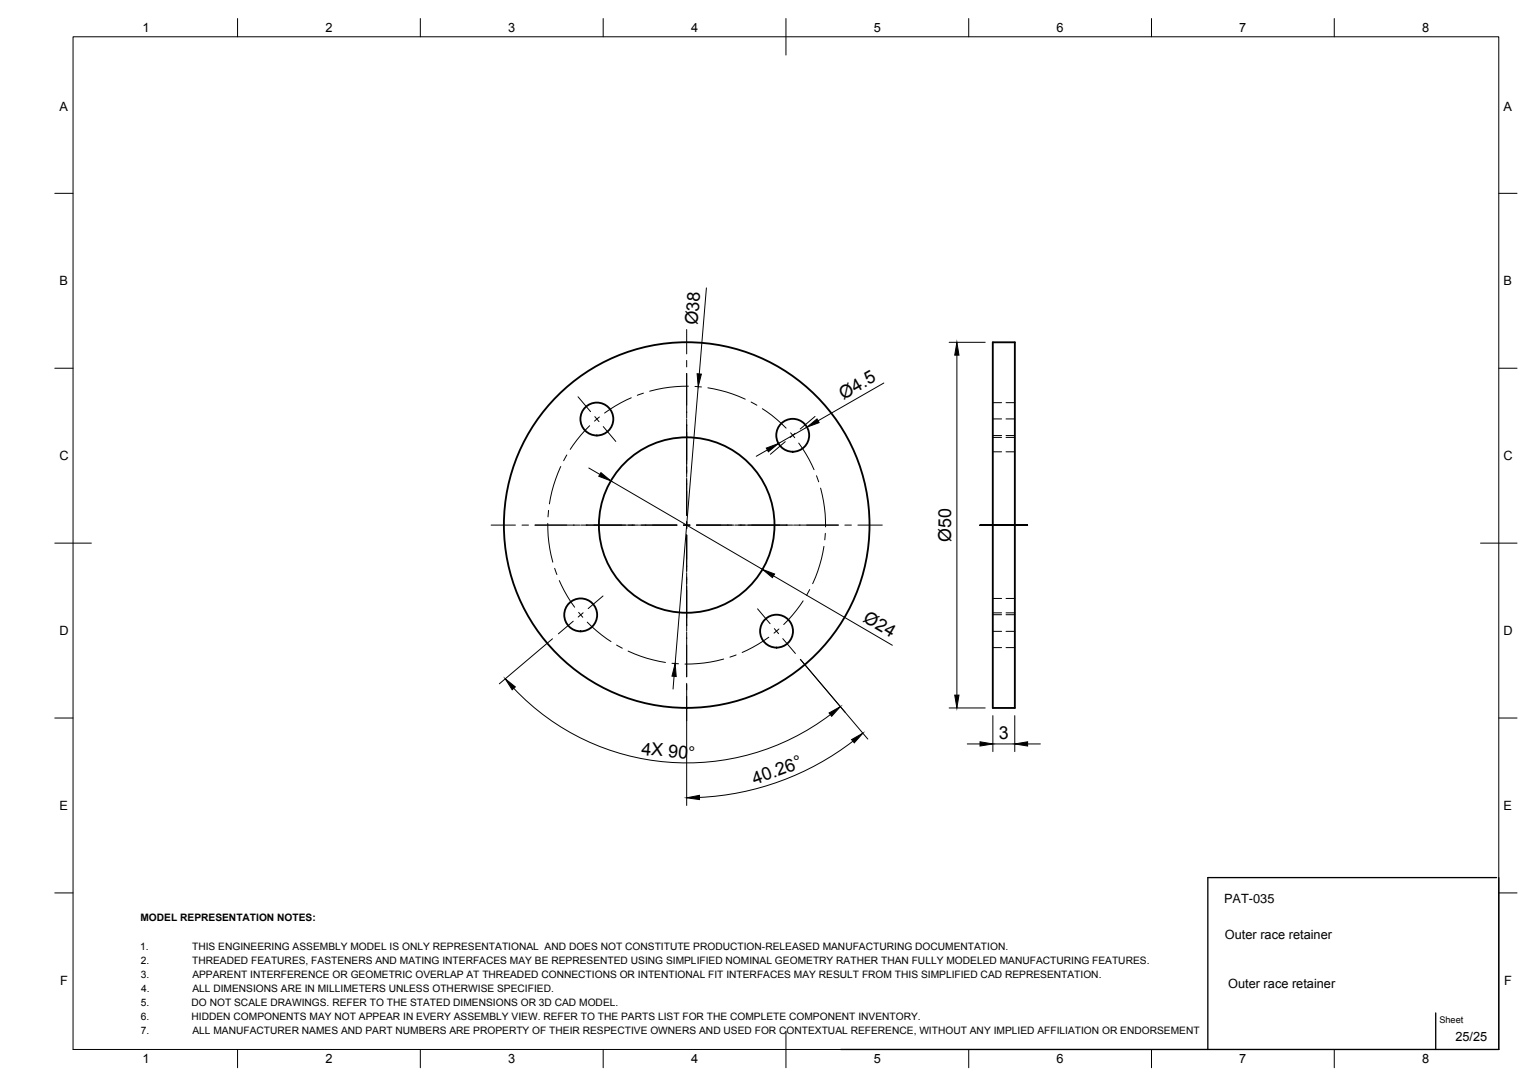
ISO-10303-21;
HEADER;
/* Generated by software containing ST-Developer
 * from STEP Tools, Inc. (www.steptools.com) 
 */

FILE_DESCRIPTION(
/* description */ ('Five-roller gravity conveyor'),
/* implementation_level */ '2;1');

FILE_NAME(
/* name */ 'Outer race retainer.step',
/* time_stamp */ '2026-10-29T15:36:43-07:00',
/* author */ (''),
/* organization */ (''),
/* preprocessor_version */ 'ST-DEVELOPER v20.2',
/* originating_system */ 'Autodesk Translation Framework v15.17.0.0',
/* authorisation */ '');

FILE_SCHEMA (('AUTOMOTIVE_DESIGN { 1 0 10303 214 3 1 1 }'));
ENDSEC;

DATA;
#10=MECHANICAL_DESIGN_GEOMETRIC_PRESENTATION_REPRESENTATION('',(#336),#7806);
#292=SHAPE_REPRESENTATION_RELATIONSHIP('SRR','None',#7931,#310);
#310=ADVANCED_BREP_SHAPE_REPRESENTATION('',(#361),#7804);
#336=STYLED_ITEM('',(#8091),#361);
#361=MANIFOLD_SOLID_BREP('Body1',#4224);
#410=FACE_BOUND('',#1146,.T.);
#411=FACE_BOUND('',#1147,.T.);
#412=FACE_BOUND('',#1148,.T.);
#413=FACE_BOUND('',#1149,.T.);
#414=FACE_BOUND('',#1150,.T.);
#415=FACE_BOUND('',#1152,.T.);
#416=FACE_BOUND('',#1153,.T.);
#417=FACE_BOUND('',#1154,.T.);
#418=FACE_BOUND('',#1155,.T.);
#419=FACE_BOUND('',#1156,.T.);
#574=CIRCLE('',#4816,0.225);
#575=CIRCLE('',#4817,0.225);
#576=CIRCLE('',#4819,0.225);
#577=CIRCLE('',#4820,0.225);
#578=CIRCLE('',#4822,0.225);
#579=CIRCLE('',#4823,0.225);
#580=CIRCLE('',#4825,0.225);
#581=CIRCLE('',#4826,0.225);
#582=CIRCLE('',#4828,1.2);
#583=CIRCLE('',#4829,1.2);
#584=CIRCLE('',#4831,2.5);
#585=CIRCLE('',#4832,2.5);
#644=CYLINDRICAL_SURFACE('',#4815,0.225);
#645=CYLINDRICAL_SURFACE('',#4818,0.225);
#646=CYLINDRICAL_SURFACE('',#4821,0.225);
#647=CYLINDRICAL_SURFACE('',#4824,0.225);
#648=CYLINDRICAL_SURFACE('',#4827,1.2);
#649=CYLINDRICAL_SURFACE('',#4830,2.5);
#859=FACE_OUTER_BOUND('',#1139,.T.);
#860=FACE_OUTER_BOUND('',#1140,.T.);
#861=FACE_OUTER_BOUND('',#1141,.T.);
#862=FACE_OUTER_BOUND('',#1142,.T.);
#863=FACE_OUTER_BOUND('',#1143,.T.);
#864=FACE_OUTER_BOUND('',#1144,.T.);
#865=FACE_OUTER_BOUND('',#1145,.T.);
#866=FACE_OUTER_BOUND('',#1151,.T.);
#1139=EDGE_LOOP('',(#3722,#3723,#3724,#3725));
#1140=EDGE_LOOP('',(#3726,#3727,#3728,#3729));
#1141=EDGE_LOOP('',(#3730,#3731,#3732,#3733));
#1142=EDGE_LOOP('',(#3734,#3735,#3736,#3737));
#1143=EDGE_LOOP('',(#3738,#3739,#3740,#3741));
#1144=EDGE_LOOP('',(#3742,#3743,#3744,#3745));
#1145=EDGE_LOOP('',(#3746));
#1146=EDGE_LOOP('',(#3747));
#1147=EDGE_LOOP('',(#3748));
#1148=EDGE_LOOP('',(#3749));
#1149=EDGE_LOOP('',(#3750));
#1150=EDGE_LOOP('',(#3751));
#1151=EDGE_LOOP('',(#3752));
#1152=EDGE_LOOP('',(#3753));
#1153=EDGE_LOOP('',(#3754));
#1154=EDGE_LOOP('',(#3755));
#1155=EDGE_LOOP('',(#3756));
#1156=EDGE_LOOP('',(#3757));
#1486=LINE('',#7607,#1827);
#1487=LINE('',#7613,#1828);
#1488=LINE('',#7619,#1829);
#1489=LINE('',#7625,#1830);
#1490=LINE('',#7631,#1831);
#1491=LINE('',#7637,#1832);
#1827=VECTOR('',#6002,0.225);
#1828=VECTOR('',#6009,0.225);
#1829=VECTOR('',#6016,0.225);
#1830=VECTOR('',#6023,0.225);
#1831=VECTOR('',#6030,1.2);
#1832=VECTOR('',#6037,2.5);
#2188=VERTEX_POINT('',#7604);
#2189=VERTEX_POINT('',#7606);
#2190=VERTEX_POINT('',#7610);
#2191=VERTEX_POINT('',#7612);
#2192=VERTEX_POINT('',#7616);
#2193=VERTEX_POINT('',#7618);
#2194=VERTEX_POINT('',#7622);
#2195=VERTEX_POINT('',#7624);
#2196=VERTEX_POINT('',#7628);
#2197=VERTEX_POINT('',#7630);
#2198=VERTEX_POINT('',#7634);
#2199=VERTEX_POINT('',#7636);
#2704=EDGE_CURVE('',#2188,#2188,#574,.T.);
#2705=EDGE_CURVE('',#2188,#2189,#1486,.T.);
#2706=EDGE_CURVE('',#2189,#2189,#575,.T.);
#2707=EDGE_CURVE('',#2190,#2190,#576,.T.);
#2708=EDGE_CURVE('',#2190,#2191,#1487,.T.);
#2709=EDGE_CURVE('',#2191,#2191,#577,.T.);
#2710=EDGE_CURVE('',#2192,#2192,#578,.T.);
#2711=EDGE_CURVE('',#2192,#2193,#1488,.T.);
#2712=EDGE_CURVE('',#2193,#2193,#579,.T.);
#2713=EDGE_CURVE('',#2194,#2194,#580,.T.);
#2714=EDGE_CURVE('',#2194,#2195,#1489,.T.);
#2715=EDGE_CURVE('',#2195,#2195,#581,.T.);
#2716=EDGE_CURVE('',#2196,#2196,#582,.T.);
#2717=EDGE_CURVE('',#2196,#2197,#1490,.T.);
#2718=EDGE_CURVE('',#2197,#2197,#583,.T.);
#2719=EDGE_CURVE('',#2198,#2198,#584,.T.);
#2720=EDGE_CURVE('',#2198,#2199,#1491,.T.);
#2721=EDGE_CURVE('',#2199,#2199,#585,.T.);
#3722=ORIENTED_EDGE('',*,*,#2704,.F.);
#3723=ORIENTED_EDGE('',*,*,#2705,.T.);
#3724=ORIENTED_EDGE('',*,*,#2706,.F.);
#3725=ORIENTED_EDGE('',*,*,#2705,.F.);
#3726=ORIENTED_EDGE('',*,*,#2707,.F.);
#3727=ORIENTED_EDGE('',*,*,#2708,.T.);
#3728=ORIENTED_EDGE('',*,*,#2709,.F.);
#3729=ORIENTED_EDGE('',*,*,#2708,.F.);
#3730=ORIENTED_EDGE('',*,*,#2710,.F.);
#3731=ORIENTED_EDGE('',*,*,#2711,.T.);
#3732=ORIENTED_EDGE('',*,*,#2712,.F.);
#3733=ORIENTED_EDGE('',*,*,#2711,.F.);
#3734=ORIENTED_EDGE('',*,*,#2713,.F.);
#3735=ORIENTED_EDGE('',*,*,#2714,.T.);
#3736=ORIENTED_EDGE('',*,*,#2715,.F.);
#3737=ORIENTED_EDGE('',*,*,#2714,.F.);
#3738=ORIENTED_EDGE('',*,*,#2716,.F.);
#3739=ORIENTED_EDGE('',*,*,#2717,.T.);
#3740=ORIENTED_EDGE('',*,*,#2718,.T.);
#3741=ORIENTED_EDGE('',*,*,#2717,.F.);
#3742=ORIENTED_EDGE('',*,*,#2719,.F.);
#3743=ORIENTED_EDGE('',*,*,#2720,.T.);
#3744=ORIENTED_EDGE('',*,*,#2721,.T.);
#3745=ORIENTED_EDGE('',*,*,#2720,.F.);
#3746=ORIENTED_EDGE('',*,*,#2719,.T.);
#3747=ORIENTED_EDGE('',*,*,#2716,.T.);
#3748=ORIENTED_EDGE('',*,*,#2715,.T.);
#3749=ORIENTED_EDGE('',*,*,#2712,.T.);
#3750=ORIENTED_EDGE('',*,*,#2709,.T.);
#3751=ORIENTED_EDGE('',*,*,#2706,.T.);
#3752=ORIENTED_EDGE('',*,*,#2721,.F.);
#3753=ORIENTED_EDGE('',*,*,#2718,.F.);
#3754=ORIENTED_EDGE('',*,*,#2713,.T.);
#3755=ORIENTED_EDGE('',*,*,#2710,.T.);
#3756=ORIENTED_EDGE('',*,*,#2707,.T.);
#3757=ORIENTED_EDGE('',*,*,#2704,.T.);
#3954=PLANE('',#4833);
#3955=PLANE('',#4834);
#4174=ADVANCED_FACE('',(#859),#644,.F.);
#4175=ADVANCED_FACE('',(#860),#645,.F.);
#4176=ADVANCED_FACE('',(#861),#646,.F.);
#4177=ADVANCED_FACE('',(#862),#647,.F.);
#4178=ADVANCED_FACE('',(#863),#648,.F.);
#4179=ADVANCED_FACE('',(#864),#649,.T.);
#4180=ADVANCED_FACE('',(#865,#410,#411,#412,#413,#414),#3954,.T.);
#4181=ADVANCED_FACE('',(#866,#415,#416,#417,#418,#419),#3955,.F.);
#4224=CLOSED_SHELL('',(#4174,#4175,#4176,#4177,#4178,#4179,#4180,#4181));
#4814=AXIS2_PLACEMENT_3D('',#7602,#5996,#5997);
#4815=AXIS2_PLACEMENT_3D('',#7603,#5998,#5999);
#4816=AXIS2_PLACEMENT_3D('',#7605,#6000,#6001);
#4817=AXIS2_PLACEMENT_3D('',#7608,#6003,#6004);
#4818=AXIS2_PLACEMENT_3D('',#7609,#6005,#6006);
#4819=AXIS2_PLACEMENT_3D('',#7611,#6007,#6008);
#4820=AXIS2_PLACEMENT_3D('',#7614,#6010,#6011);
#4821=AXIS2_PLACEMENT_3D('',#7615,#6012,#6013);
#4822=AXIS2_PLACEMENT_3D('',#7617,#6014,#6015);
#4823=AXIS2_PLACEMENT_3D('',#7620,#6017,#6018);
#4824=AXIS2_PLACEMENT_3D('',#7621,#6019,#6020);
#4825=AXIS2_PLACEMENT_3D('',#7623,#6021,#6022);
#4826=AXIS2_PLACEMENT_3D('',#7626,#6024,#6025);
#4827=AXIS2_PLACEMENT_3D('',#7627,#6026,#6027);
#4828=AXIS2_PLACEMENT_3D('',#7629,#6028,#6029);
#4829=AXIS2_PLACEMENT_3D('',#7632,#6031,#6032);
#4830=AXIS2_PLACEMENT_3D('',#7633,#6033,#6034);
#4831=AXIS2_PLACEMENT_3D('',#7635,#6035,#6036);
#4832=AXIS2_PLACEMENT_3D('',#7638,#6038,#6039);
#4833=AXIS2_PLACEMENT_3D('',#7639,#6040,#6041);
#4834=AXIS2_PLACEMENT_3D('',#7640,#6042,#6043);
#5996=DIRECTION('axis',(0.,0.,1.));
#5997=DIRECTION('refdir',(1.,0.,0.));
#5998=DIRECTION('center_axis',(0.,1.,0.));
#5999=DIRECTION('ref_axis',(1.,0.,0.));
#6000=DIRECTION('center_axis',(0.,1.,0.));
#6001=DIRECTION('ref_axis',(1.,0.,0.));
#6002=DIRECTION('',(0.,1.,0.));
#6003=DIRECTION('center_axis',(0.,-1.,0.));
#6004=DIRECTION('ref_axis',(1.,0.,0.));
#6005=DIRECTION('center_axis',(0.,1.,0.));
#6006=DIRECTION('ref_axis',(1.,0.,0.));
#6007=DIRECTION('center_axis',(0.,1.,0.));
#6008=DIRECTION('ref_axis',(1.,0.,0.));
#6009=DIRECTION('',(0.,1.,0.));
#6010=DIRECTION('center_axis',(0.,-1.,0.));
#6011=DIRECTION('ref_axis',(1.,0.,0.));
#6012=DIRECTION('center_axis',(0.,1.,0.));
#6013=DIRECTION('ref_axis',(1.,0.,0.));
#6014=DIRECTION('center_axis',(0.,1.,0.));
#6015=DIRECTION('ref_axis',(1.,0.,0.));
#6016=DIRECTION('',(0.,1.,0.));
#6017=DIRECTION('center_axis',(0.,-1.,0.));
#6018=DIRECTION('ref_axis',(1.,0.,0.));
#6019=DIRECTION('center_axis',(0.,1.,0.));
#6020=DIRECTION('ref_axis',(1.,0.,0.));
#6021=DIRECTION('center_axis',(0.,1.,0.));
#6022=DIRECTION('ref_axis',(1.,0.,0.));
#6023=DIRECTION('',(0.,1.,0.));
#6024=DIRECTION('center_axis',(0.,-1.,0.));
#6025=DIRECTION('ref_axis',(1.,0.,0.));
#6026=DIRECTION('center_axis',(0.,1.,0.));
#6027=DIRECTION('ref_axis',(1.,0.,0.));
#6028=DIRECTION('center_axis',(0.,-1.,0.));
#6029=DIRECTION('ref_axis',(1.,0.,0.));
#6030=DIRECTION('',(0.,-1.,0.));
#6031=DIRECTION('center_axis',(0.,-1.,0.));
#6032=DIRECTION('ref_axis',(1.,0.,0.));
#6033=DIRECTION('center_axis',(0.,1.,0.));
#6034=DIRECTION('ref_axis',(1.,0.,0.));
#6035=DIRECTION('center_axis',(0.,1.,0.));
#6036=DIRECTION('ref_axis',(1.,0.,0.));
#6037=DIRECTION('',(0.,-1.,0.));
#6038=DIRECTION('center_axis',(0.,1.,0.));
#6039=DIRECTION('ref_axis',(1.,0.,0.));
#6040=DIRECTION('center_axis',(0.,1.,0.));
#6041=DIRECTION('ref_axis',(1.,0.,0.));
#6042=DIRECTION('center_axis',(0.,1.,0.));
#6043=DIRECTION('ref_axis',(1.,0.,0.));
#7602=CARTESIAN_POINT('',(0.,0.,0.));
#7603=CARTESIAN_POINT('Origin',(-1.9,-0.4,4.5));
#7604=CARTESIAN_POINT('',(-2.125,-0.3,4.5));
#7605=CARTESIAN_POINT('Origin',(-1.9,-0.3,4.5));
#7606=CARTESIAN_POINT('',(-2.125,0.,4.5));
#7607=CARTESIAN_POINT('',(-2.125,-0.4,4.5));
#7608=CARTESIAN_POINT('Origin',(-1.9,0.,4.5));
#7609=CARTESIAN_POINT('Origin',(1.16341445918999E-16,-0.4,6.4));
#7610=CARTESIAN_POINT('',(-0.225,-0.3,6.4));
#7611=CARTESIAN_POINT('Origin',(1.16341445918999E-16,-0.3,6.4));
#7612=CARTESIAN_POINT('',(-0.225,0.,6.4));
#7613=CARTESIAN_POINT('',(-0.225,-0.4,6.4));
#7614=CARTESIAN_POINT('Origin',(1.16341445918999E-16,0.,6.4));
#7615=CARTESIAN_POINT('Origin',(1.9,-0.4,4.5));
#7616=CARTESIAN_POINT('',(1.675,-0.3,4.5));
#7617=CARTESIAN_POINT('Origin',(1.9,-0.3,4.5));
#7618=CARTESIAN_POINT('',(1.675,0.,4.5));
#7619=CARTESIAN_POINT('',(1.675,-0.4,4.5));
#7620=CARTESIAN_POINT('Origin',(1.9,0.,4.5));
#7621=CARTESIAN_POINT('Origin',(-3.49024337756996E-16,-0.4,2.6));
#7622=CARTESIAN_POINT('',(-0.225,-0.3,2.6));
#7623=CARTESIAN_POINT('Origin',(-3.49024337756996E-16,-0.3,2.6));
#7624=CARTESIAN_POINT('',(-0.225,0.,2.6));
#7625=CARTESIAN_POINT('',(-0.225,-0.4,2.6));
#7626=CARTESIAN_POINT('Origin',(-3.49024337756996E-16,0.,2.6));
#7627=CARTESIAN_POINT('Origin',(0.,-0.3,4.5));
#7628=CARTESIAN_POINT('',(-1.2,0.,4.5));
#7629=CARTESIAN_POINT('Origin',(0.,0.,4.5));
#7630=CARTESIAN_POINT('',(-1.2,-0.3,4.5));
#7631=CARTESIAN_POINT('',(-1.2,-0.3,4.5));
#7632=CARTESIAN_POINT('Origin',(0.,-0.3,4.5));
#7633=CARTESIAN_POINT('Origin',(0.,-0.3,4.5));
#7634=CARTESIAN_POINT('',(-2.5,0.,4.5));
#7635=CARTESIAN_POINT('Origin',(0.,0.,4.5));
#7636=CARTESIAN_POINT('',(-2.5,-0.3,4.5));
#7637=CARTESIAN_POINT('',(-2.5,-0.3,4.5));
#7638=CARTESIAN_POINT('Origin',(0.,-0.3,4.5));
#7639=CARTESIAN_POINT('Origin',(0.,0.,4.5));
#7640=CARTESIAN_POINT('Origin',(0.,-0.3,4.5));
#7780=UNCERTAINTY_MEASURE_WITH_UNIT(LENGTH_MEASURE(0.001),#7807,
'DISTANCE_ACCURACY_VALUE',
'Maximum model space distance between geometric entities at asserted c
onnectivities');
#7782=UNCERTAINTY_MEASURE_WITH_UNIT(LENGTH_MEASURE(0.001),#7807,
'DISTANCE_ACCURACY_VALUE',
'Maximum model space distance between geometric entities at asserted c
onnectivities');
#7804=(
GEOMETRIC_REPRESENTATION_CONTEXT(3)
GLOBAL_UNCERTAINTY_ASSIGNED_CONTEXT((#7780))
GLOBAL_UNIT_ASSIGNED_CONTEXT((#7807,#7809,#7810))
REPRESENTATION_CONTEXT('','3D')
);
#7806=(
GEOMETRIC_REPRESENTATION_CONTEXT(3)
GLOBAL_UNCERTAINTY_ASSIGNED_CONTEXT((#7782))
GLOBAL_UNIT_ASSIGNED_CONTEXT((#7807,#7809,#7810))
REPRESENTATION_CONTEXT('','3D')
);
#7807=(
LENGTH_UNIT()
NAMED_UNIT(*)
SI_UNIT(.CENTI.,.METRE.)
);
#7809=(
NAMED_UNIT(*)
PLANE_ANGLE_UNIT()
SI_UNIT($,.RADIAN.)
);
#7810=(
NAMED_UNIT(*)
SI_UNIT($,.STERADIAN.)
SOLID_ANGLE_UNIT()
);
#7832=SHAPE_DEFINITION_REPRESENTATION(#7860,#7931);
#7860=PRODUCT_DEFINITION_SHAPE('',$,#7955);
#7931=SHAPE_REPRESENTATION('',(#4814),#7804);
#7933=PRODUCT_DEFINITION_CONTEXT('part definition',#8004,'design');
#7955=PRODUCT_DEFINITION('Outer race retainer','Outer race retainer',#7978,
#7933);
#7978=PRODUCT_DEFINITION_FORMATION('',$,#8027);
#8004=APPLICATION_CONTEXT(
'Core Data for Automotive Mechanical Design Process');
#8005=PRODUCT_CONTEXT('part definition',#8004,'mechanical');
#8027=PRODUCT('Outer race retainer','Outer race retainer',
'Outer race retainer',(#8005));
#8085=COLOUR_RGB('Grey',0.48,0.52,0.57);
#8086=FILL_AREA_STYLE_COLOUR('',#8085);
#8087=FILL_AREA_STYLE('',(#8086));
#8088=SURFACE_STYLE_FILL_AREA(#8087);
#8089=SURFACE_SIDE_STYLE('',(#8088));
#8090=SURFACE_STYLE_USAGE(.BOTH.,#8089);
#8091=PRESENTATION_STYLE_ASSIGNMENT((#8090));
ENDSEC;
END-ISO-10303-21;
